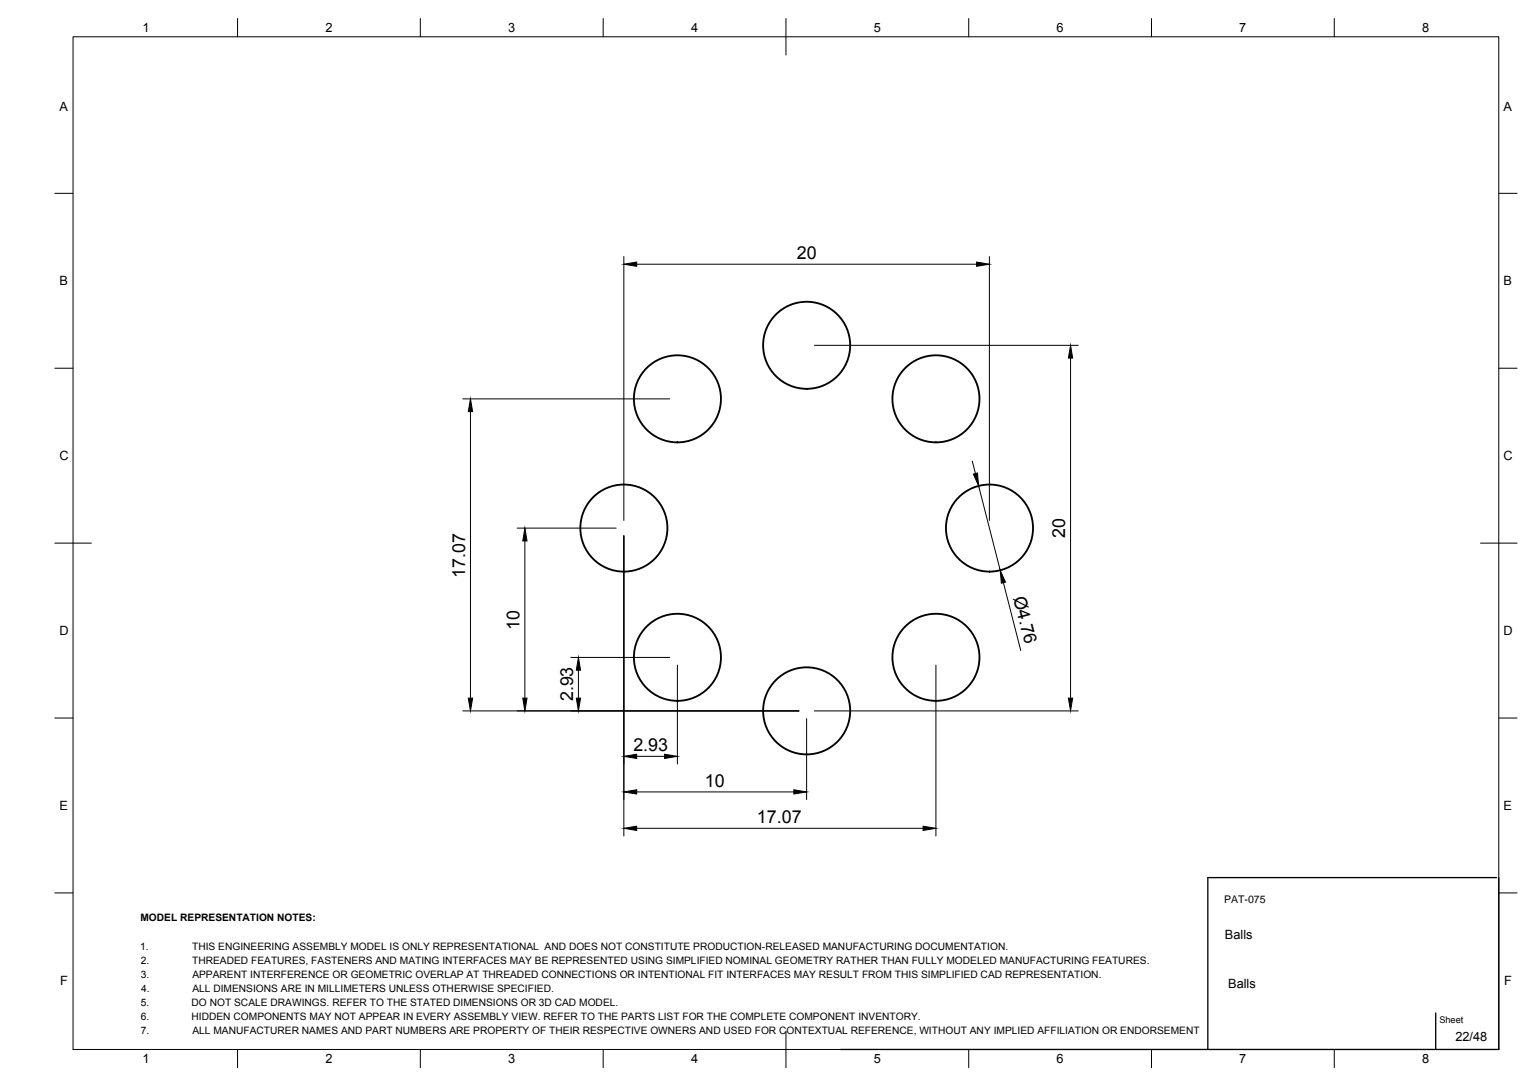
ISO-10303-21;
HEADER;
/* Generated by software containing ST-Developer
 * from STEP Tools, Inc. (www.steptools.com) 
 */

FILE_DESCRIPTION(
/* description */ ('Over-Centre Plunger Toggle Clamp on Slotted Fixture Frame'),
/* implementation_level */ '2;1');

FILE_NAME(
/* name */ 
'Balls.step',
/* time_stamp */ '2026-10-28T03:23:24-07:00',
/* author */ (''),
/* organization */ (''),
/* preprocessor_version */ 'ST-DEVELOPER v20.2',
/* originating_system */ 'Autodesk Translation Framework v15.17.0.0',
/* authorisation */ '');

FILE_SCHEMA (('AUTOMOTIVE_DESIGN { 1 0 10303 214 3 1 1 }'));
ENDSEC;

DATA;
#10=MECHANICAL_DESIGN_GEOMETRIC_PRESENTATION_REPRESENTATION('',(#531,#532,#533,#534,#535,#536,#537,#538),#15212);
#379=SPHERICAL_SURFACE('',#9206,0.23815);
#380=SPHERICAL_SURFACE('',#9208,0.23815);
#381=SPHERICAL_SURFACE('',#9210,0.23815);
#382=SPHERICAL_SURFACE('',#9212,0.23815);
#383=SPHERICAL_SURFACE('',#9214,0.23815);
#384=SPHERICAL_SURFACE('',#9216,0.23815);
#385=SPHERICAL_SURFACE('',#9218,0.23815);
#386=SPHERICAL_SURFACE('',#9220,0.23815);
#447=SHAPE_REPRESENTATION_RELATIONSHIP('SRR','None',#15422,#489);
#489=ADVANCED_BREP_SHAPE_REPRESENTATION('',(#581,#582,#583,#584,#585,#586,
#587,#588),#15184);
#531=STYLED_ITEM('',(#15719),#581);
#532=STYLED_ITEM('',(#15719),#582);
#533=STYLED_ITEM('',(#15719),#583);
#534=STYLED_ITEM('',(#15719),#584);
#535=STYLED_ITEM('',(#15719),#585);
#536=STYLED_ITEM('',(#15719),#586);
#537=STYLED_ITEM('',(#15719),#587);
#538=STYLED_ITEM('',(#15719),#588);
#581=MANIFOLD_SOLID_BREP('Body1',#8264);
#582=MANIFOLD_SOLID_BREP('Body2',#8265);
#583=MANIFOLD_SOLID_BREP('Body3',#8266);
#584=MANIFOLD_SOLID_BREP('Body4',#8267);
#585=MANIFOLD_SOLID_BREP('Body5',#8268);
#586=MANIFOLD_SOLID_BREP('Body6',#8269);
#587=MANIFOLD_SOLID_BREP('Body7',#8270);
#588=MANIFOLD_SOLID_BREP('Body8',#8271);
#1334=FACE_OUTER_BOUND('',#1933,.T.);
#1335=FACE_OUTER_BOUND('',#1934,.T.);
#1336=FACE_OUTER_BOUND('',#1935,.T.);
#1337=FACE_OUTER_BOUND('',#1936,.T.);
#1338=FACE_OUTER_BOUND('',#1937,.T.);
#1339=FACE_OUTER_BOUND('',#1938,.T.);
#1340=FACE_OUTER_BOUND('',#1939,.T.);
#1341=FACE_OUTER_BOUND('',#1940,.T.);
#1933=EDGE_LOOP('',(#6693,#6694));
#1934=EDGE_LOOP('',(#6695,#6696));
#1935=EDGE_LOOP('',(#6697,#6698));
#1936=EDGE_LOOP('',(#6699,#6700));
#1937=EDGE_LOOP('',(#6701,#6702));
#1938=EDGE_LOOP('',(#6703,#6704));
#1939=EDGE_LOOP('',(#6705,#6706));
#1940=EDGE_LOOP('',(#6707,#6708));
#3663=CIRCLE('',#9207,0.23815);
#3664=CIRCLE('',#9209,0.23815);
#3665=CIRCLE('',#9211,0.23815);
#3666=CIRCLE('',#9213,0.23815);
#3667=CIRCLE('',#9215,0.23815);
#3668=CIRCLE('',#9217,0.23815);
#3669=CIRCLE('',#9219,0.23815);
#3670=CIRCLE('',#9221,0.23815);
#4231=VERTEX_POINT('',#13570);
#4232=VERTEX_POINT('',#13571);
#4233=VERTEX_POINT('',#13574);
#4234=VERTEX_POINT('',#13575);
#4235=VERTEX_POINT('',#13578);
#4236=VERTEX_POINT('',#13579);
#4237=VERTEX_POINT('',#13582);
#4238=VERTEX_POINT('',#13583);
#4239=VERTEX_POINT('',#13586);
#4240=VERTEX_POINT('',#13587);
#4241=VERTEX_POINT('',#13590);
#4242=VERTEX_POINT('',#13591);
#4243=VERTEX_POINT('',#13594);
#4244=VERTEX_POINT('',#13595);
#4245=VERTEX_POINT('',#13598);
#4246=VERTEX_POINT('',#13599);
#5107=EDGE_CURVE('',#4231,#4232,#3663,.T.);
#5108=EDGE_CURVE('',#4233,#4234,#3664,.T.);
#5109=EDGE_CURVE('',#4235,#4236,#3665,.T.);
#5110=EDGE_CURVE('',#4237,#4238,#3666,.T.);
#5111=EDGE_CURVE('',#4239,#4240,#3667,.T.);
#5112=EDGE_CURVE('',#4241,#4242,#3668,.T.);
#5113=EDGE_CURVE('',#4243,#4244,#3669,.T.);
#5114=EDGE_CURVE('',#4245,#4246,#3670,.T.);
#6693=ORIENTED_EDGE('',*,*,#5107,.T.);
#6694=ORIENTED_EDGE('',*,*,#5107,.F.);
#6695=ORIENTED_EDGE('',*,*,#5108,.T.);
#6696=ORIENTED_EDGE('',*,*,#5108,.F.);
#6697=ORIENTED_EDGE('',*,*,#5109,.T.);
#6698=ORIENTED_EDGE('',*,*,#5109,.F.);
#6699=ORIENTED_EDGE('',*,*,#5110,.T.);
#6700=ORIENTED_EDGE('',*,*,#5110,.F.);
#6701=ORIENTED_EDGE('',*,*,#5111,.T.);
#6702=ORIENTED_EDGE('',*,*,#5111,.F.);
#6703=ORIENTED_EDGE('',*,*,#5112,.T.);
#6704=ORIENTED_EDGE('',*,*,#5112,.F.);
#6705=ORIENTED_EDGE('',*,*,#5113,.T.);
#6706=ORIENTED_EDGE('',*,*,#5113,.F.);
#6707=ORIENTED_EDGE('',*,*,#5114,.T.);
#6708=ORIENTED_EDGE('',*,*,#5114,.F.);
#8006=ADVANCED_FACE('',(#1334),#379,.T.);
#8007=ADVANCED_FACE('',(#1335),#380,.T.);
#8008=ADVANCED_FACE('',(#1336),#381,.T.);
#8009=ADVANCED_FACE('',(#1337),#382,.T.);
#8010=ADVANCED_FACE('',(#1338),#383,.T.);
#8011=ADVANCED_FACE('',(#1339),#384,.T.);
#8012=ADVANCED_FACE('',(#1340),#385,.T.);
#8013=ADVANCED_FACE('',(#1341),#386,.T.);
#8264=CLOSED_SHELL('',(#8006));
#8265=CLOSED_SHELL('',(#8007));
#8266=CLOSED_SHELL('',(#8008));
#8267=CLOSED_SHELL('',(#8009));
#8268=CLOSED_SHELL('',(#8010));
#8269=CLOSED_SHELL('',(#8011));
#8270=CLOSED_SHELL('',(#8012));
#8271=CLOSED_SHELL('',(#8013));
#9205=AXIS2_PLACEMENT_3D('',#13568,#11026,#11027);
#9206=AXIS2_PLACEMENT_3D('',#13569,#11028,#11029);
#9207=AXIS2_PLACEMENT_3D('',#13572,#11030,#11031);
#9208=AXIS2_PLACEMENT_3D('',#13573,#11032,#11033);
#9209=AXIS2_PLACEMENT_3D('',#13576,#11034,#11035);
#9210=AXIS2_PLACEMENT_3D('',#13577,#11036,#11037);
#9211=AXIS2_PLACEMENT_3D('',#13580,#11038,#11039);
#9212=AXIS2_PLACEMENT_3D('',#13581,#11040,#11041);
#9213=AXIS2_PLACEMENT_3D('',#13584,#11042,#11043);
#9214=AXIS2_PLACEMENT_3D('',#13585,#11044,#11045);
#9215=AXIS2_PLACEMENT_3D('',#13588,#11046,#11047);
#9216=AXIS2_PLACEMENT_3D('',#13589,#11048,#11049);
#9217=AXIS2_PLACEMENT_3D('',#13592,#11050,#11051);
#9218=AXIS2_PLACEMENT_3D('',#13593,#11052,#11053);
#9219=AXIS2_PLACEMENT_3D('',#13596,#11054,#11055);
#9220=AXIS2_PLACEMENT_3D('',#13597,#11056,#11057);
#9221=AXIS2_PLACEMENT_3D('',#13600,#11058,#11059);
#11026=DIRECTION('axis',(0.,0.,1.));
#11027=DIRECTION('refdir',(1.,0.,0.));
#11028=DIRECTION('center_axis',(0.,0.,1.));
#11029=DIRECTION('ref_axis',(1.,0.,0.));
#11030=DIRECTION('center_axis',(1.22464679914735E-16,-1.,0.));
#11031=DIRECTION('ref_axis',(-1.,-1.22464679914735E-16,0.));
#11032=DIRECTION('center_axis',(0.707106781186548,0.,0.707106781186548));
#11033=DIRECTION('ref_axis',(0.707106781186548,0.,-0.707106781186548));
#11034=DIRECTION('center_axis',(8.65956056235494E-17,-1.,-8.65956056235493E-17));
#11035=DIRECTION('ref_axis',(-0.707106781186547,-1.22464679914735E-16,0.707106781186547));
#11036=DIRECTION('center_axis',(1.,0.,0.));
#11037=DIRECTION('ref_axis',(6.12323399573676E-17,0.,-1.));
#11038=DIRECTION('center_axis',(7.49879891330929E-33,-1.,-1.22464679914735E-16));
#11039=DIRECTION('ref_axis',(-6.12323399573676E-17,-1.22464679914735E-16,
1.));
#11040=DIRECTION('center_axis',(0.707106781186548,0.,-0.707106781186548));
#11041=DIRECTION('ref_axis',(-0.707106781186548,0.,-0.707106781186548));
#11042=DIRECTION('center_axis',(-8.65956056235493E-17,-1.,-8.65956056235494E-17));
#11043=DIRECTION('ref_axis',(0.707106781186547,-1.22464679914735E-16,0.707106781186547));
#11044=DIRECTION('center_axis',(0.,0.,-1.));
#11045=DIRECTION('ref_axis',(-1.,0.,-1.22464679914735E-16));
#11046=DIRECTION('center_axis',(-1.22464679914735E-16,-1.,-1.49975978266186E-32));
#11047=DIRECTION('ref_axis',(1.,-1.22464679914735E-16,1.22464679914735E-16));
#11048=DIRECTION('center_axis',(-0.707106781186547,0.,-0.707106781186548));
#11049=DIRECTION('ref_axis',(-0.707106781186548,0.,0.707106781186547));
#11050=DIRECTION('center_axis',(-8.65956056235493E-17,-1.,8.65956056235493E-17));
#11051=DIRECTION('ref_axis',(0.707106781186548,-1.22464679914735E-16,-0.707106781186547));
#11052=DIRECTION('center_axis',(-1.,0.,0.));
#11053=DIRECTION('ref_axis',(-1.83697019872103E-16,0.,1.));
#11054=DIRECTION('center_axis',(-2.24963967399279E-32,-1.,1.22464679914735E-16));
#11055=DIRECTION('ref_axis',(1.83697019872103E-16,-1.22464679914735E-16,
-1.));
#11056=DIRECTION('center_axis',(-0.707106781186548,0.,0.707106781186548));
#11057=DIRECTION('ref_axis',(0.707106781186547,0.,0.707106781186548));
#11058=DIRECTION('center_axis',(8.65956056235493E-17,-1.,8.65956056235493E-17));
#11059=DIRECTION('ref_axis',(-0.707106781186547,-1.22464679914735E-16,-0.707106781186548));
#13568=CARTESIAN_POINT('',(0.,0.,0.));
#13569=CARTESIAN_POINT('Origin',(1.,0.,0.));
#13570=CARTESIAN_POINT('',(1.,-1.78583896120461E-33,0.23815));
#13571=CARTESIAN_POINT('',(1.,-1.78583896120461E-33,-0.23815));
#13572=CARTESIAN_POINT('Origin',(1.,0.,0.));
#13573=CARTESIAN_POINT('Origin',(0.707106781186548,0.,-0.707106781186547));
#13574=CARTESIAN_POINT('',(0.875504261126124,-1.78583896120461E-33,-0.538709301246971));
#13575=CARTESIAN_POINT('',(0.538709301246971,-1.78583896120461E-33,-0.875504261126124));
#13576=CARTESIAN_POINT('Origin',(0.707106781186548,0.,-0.707106781186547));
#13577=CARTESIAN_POINT('Origin',(6.12323399573677E-17,0.,-1.));
#13578=CARTESIAN_POINT('',(0.23815,-1.78583896120461E-33,-1.));
#13579=CARTESIAN_POINT('',(-0.23815,-1.78583896120461E-33,-1.));
#13580=CARTESIAN_POINT('Origin',(6.12323399573677E-17,0.,-1.));
#13581=CARTESIAN_POINT('Origin',(-0.707106781186547,0.,-0.707106781186548));
#13582=CARTESIAN_POINT('',(-0.538709301246971,-1.78583896120461E-33,-0.875504261126124));
#13583=CARTESIAN_POINT('',(-0.875504261126124,-1.78583896120461E-33,-0.538709301246971));
#13584=CARTESIAN_POINT('Origin',(-0.707106781186547,0.,-0.707106781186548));
#13585=CARTESIAN_POINT('Origin',(-1.,0.,-1.22464679914735E-16));
#13586=CARTESIAN_POINT('',(-1.,-1.78583896120461E-33,-0.23815));
#13587=CARTESIAN_POINT('',(-1.,-1.78583896120461E-33,0.23815));
#13588=CARTESIAN_POINT('Origin',(-1.,0.,-1.22464679914735E-16));
#13589=CARTESIAN_POINT('Origin',(-0.707106781186548,0.,0.707106781186547));
#13590=CARTESIAN_POINT('',(-0.875504261126124,-7.94881478324376E-33,0.538709301246971));
#13591=CARTESIAN_POINT('',(-0.538709301246971,4.37713686083455E-33,0.875504261126124));
#13592=CARTESIAN_POINT('Origin',(-0.707106781186548,0.,0.707106781186547));
#13593=CARTESIAN_POINT('Origin',(-1.83697019872103E-16,0.,1.));
#13594=CARTESIAN_POINT('',(-0.23815,-1.78583896120461E-33,1.));
#13595=CARTESIAN_POINT('',(0.23815,-1.78583896120461E-33,1.));
#13596=CARTESIAN_POINT('Origin',(-1.83697019872103E-16,0.,1.));
#13597=CARTESIAN_POINT('Origin',(0.707106781186547,0.,0.707106781186548));
#13598=CARTESIAN_POINT('',(0.538709301246971,-4.86732687222419E-33,0.875504261126124));
#13599=CARTESIAN_POINT('',(0.875504261126124,1.29564894981497E-33,0.538709301246971));
#13600=CARTESIAN_POINT('Origin',(0.707106781186547,0.,0.707106781186548));
#15134=UNCERTAINTY_MEASURE_WITH_UNIT(LENGTH_MEASURE(0.001),#15213,
'DISTANCE_ACCURACY_VALUE',
'Maximum model space distance between geometric entities at asserted c
onnectivities');
#15162=UNCERTAINTY_MEASURE_WITH_UNIT(LENGTH_MEASURE(0.001),#15213,
'DISTANCE_ACCURACY_VALUE',
'Maximum model space distance between geometric entities at asserted c
onnectivities');
#15184=(
GEOMETRIC_REPRESENTATION_CONTEXT(3)
GLOBAL_UNCERTAINTY_ASSIGNED_CONTEXT((#15134))
GLOBAL_UNIT_ASSIGNED_CONTEXT((#15213,#15215,#15216))
REPRESENTATION_CONTEXT('','3D')
);
#15212=(
GEOMETRIC_REPRESENTATION_CONTEXT(3)
GLOBAL_UNCERTAINTY_ASSIGNED_CONTEXT((#15162))
GLOBAL_UNIT_ASSIGNED_CONTEXT((#15213,#15215,#15216))
REPRESENTATION_CONTEXT('','3D')
);
#15213=(
LENGTH_UNIT()
NAMED_UNIT(*)
SI_UNIT(.CENTI.,.METRE.)
);
#15215=(
NAMED_UNIT(*)
PLANE_ANGLE_UNIT()
SI_UNIT($,.RADIAN.)
);
#15216=(
NAMED_UNIT(*)
SI_UNIT($,.STERADIAN.)
SOLID_ANGLE_UNIT()
);
#15238=SHAPE_DEFINITION_REPRESENTATION(#15287,#15422);
#15287=PRODUCT_DEFINITION_SHAPE('',$,#15472);
#15422=SHAPE_REPRESENTATION('',(#9205),#15184);
#15450=PRODUCT_DEFINITION_CONTEXT('part definition',#15599,'design');
#15472=PRODUCT_DEFINITION('Balls','Balls',#15521,#15450);
#15521=PRODUCT_DEFINITION_FORMATION('',$,#15622);
#15599=APPLICATION_CONTEXT(
'Core Data for Automotive Mechanical Design Process');
#15600=PRODUCT_CONTEXT('part definition',#15599,'mechanical');
#15622=PRODUCT('Balls','Balls','Balls',(#15600));
#15713=COLOUR_RGB('Grey',0.48,0.52,0.57);
#15714=FILL_AREA_STYLE_COLOUR('',#15713);
#15715=FILL_AREA_STYLE('',(#15714));
#15716=SURFACE_STYLE_FILL_AREA(#15715);
#15717=SURFACE_SIDE_STYLE('',(#15716));
#15718=SURFACE_STYLE_USAGE(.BOTH.,#15717);
#15719=PRESENTATION_STYLE_ASSIGNMENT((#15718));
ENDSEC;
END-ISO-10303-21;
